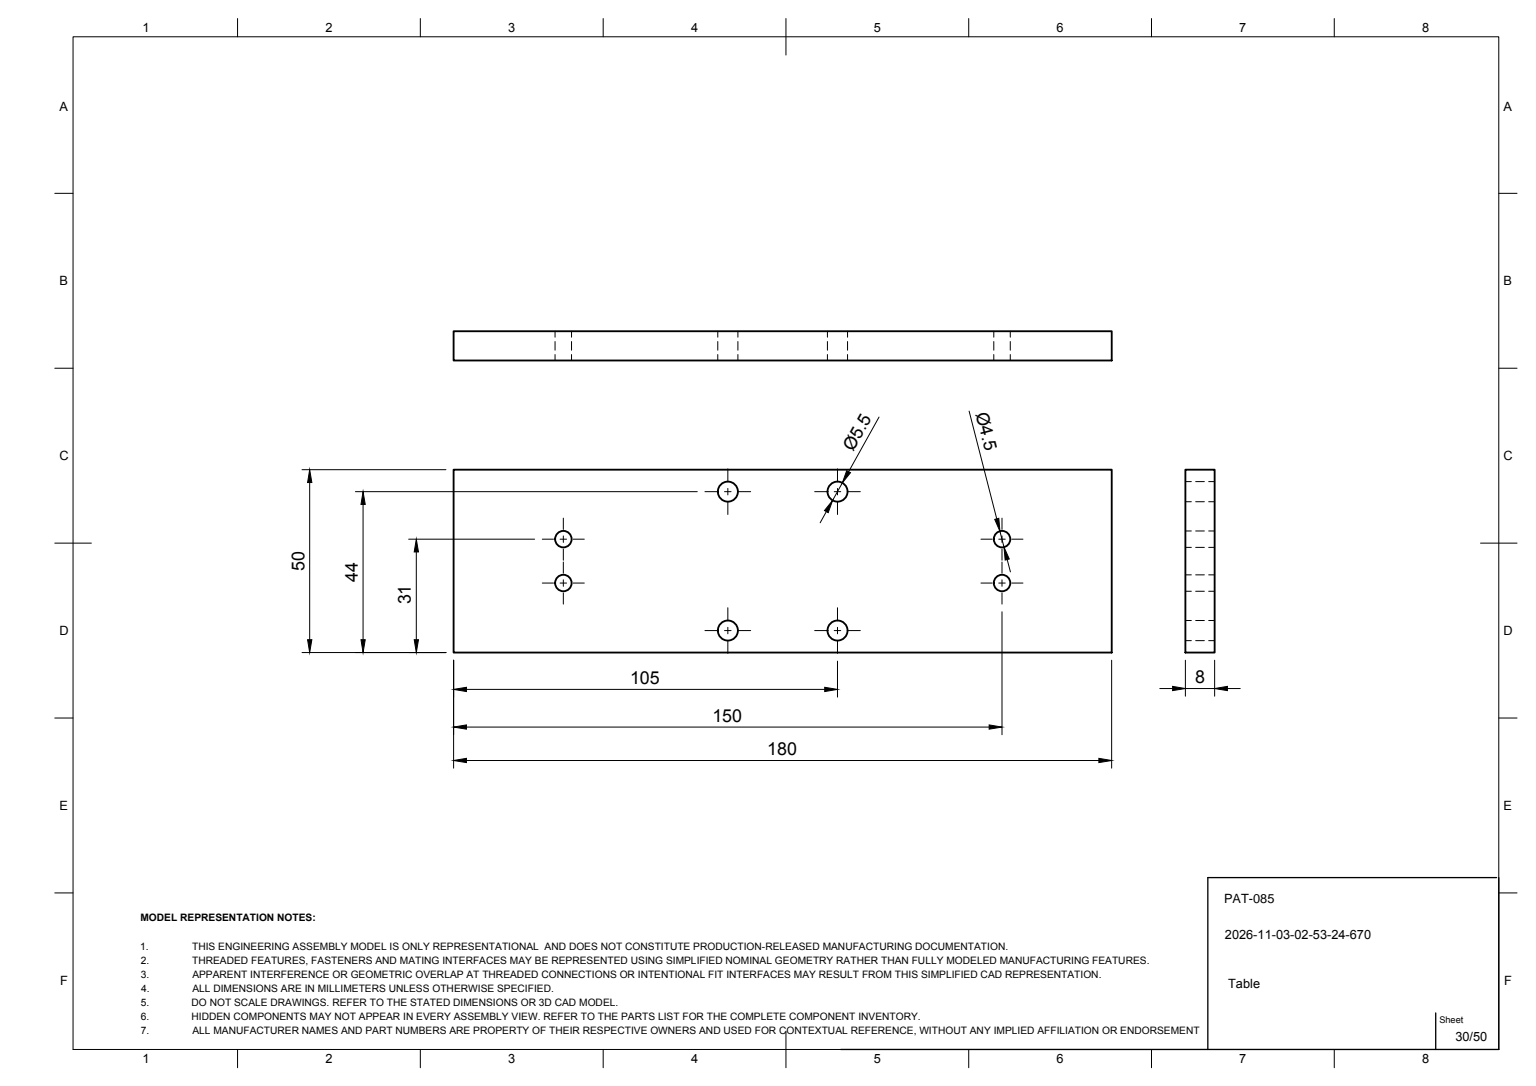
ISO-10303-21;
HEADER;
/* Generated by software containing ST-Developer
 * from STEP Tools, Inc. (www.steptools.com) 
 */

FILE_DESCRIPTION(
/* description */ ('Rack and pinion manual slide'),
/* implementation_level */ '2;1');

FILE_NAME(
/* name */ 'Table.step',
/* time_stamp */ '2026-10-28T03:22:49-07:00',
/* author */ (''),
/* organization */ (''),
/* preprocessor_version */ 'ST-DEVELOPER v20.2',
/* originating_system */ 'Autodesk Translation Framework v15.17.0.0',
/* authorisation */ '');

FILE_SCHEMA (('AUTOMOTIVE_DESIGN { 1 0 10303 214 3 1 1 }'));
ENDSEC;

DATA;
#10=MECHANICAL_DESIGN_GEOMETRIC_PRESENTATION_REPRESENTATION('',(#764),#34851);
#665=SHAPE_REPRESENTATION_RELATIONSHIP('SRR','None',#35102,#711);
#711=ADVANCED_BREP_SHAPE_REPRESENTATION('',(#815),#34827);
#764=STYLED_ITEM('',(#35425),#815);
#815=MANIFOLD_SOLID_BREP('Body1',#13786);
#985=FACE_BOUND('',#2766,.T.);
#986=FACE_BOUND('',#2767,.T.);
#987=FACE_BOUND('',#2768,.T.);
#988=FACE_BOUND('',#2769,.T.);
#989=FACE_BOUND('',#2770,.T.);
#990=FACE_BOUND('',#2771,.T.);
#991=FACE_BOUND('',#2772,.T.);
#992=FACE_BOUND('',#2773,.T.);
#993=FACE_BOUND('',#2775,.T.);
#994=FACE_BOUND('',#2776,.T.);
#995=FACE_BOUND('',#2777,.T.);
#996=FACE_BOUND('',#2778,.T.);
#997=FACE_BOUND('',#2779,.T.);
#998=FACE_BOUND('',#2780,.T.);
#999=FACE_BOUND('',#2781,.T.);
#1000=FACE_BOUND('',#2782,.T.);
#1245=PLANE('',#14956);
#1246=PLANE('',#14957);
#1247=PLANE('',#14958);
#1248=PLANE('',#14959);
#1249=PLANE('',#14960);
#1250=PLANE('',#14961);
#1862=FACE_OUTER_BOUND('',#2753,.T.);
#1863=FACE_OUTER_BOUND('',#2754,.T.);
#1864=FACE_OUTER_BOUND('',#2755,.T.);
#1865=FACE_OUTER_BOUND('',#2756,.T.);
#1866=FACE_OUTER_BOUND('',#2757,.T.);
#1867=FACE_OUTER_BOUND('',#2758,.T.);
#1868=FACE_OUTER_BOUND('',#2759,.T.);
#1869=FACE_OUTER_BOUND('',#2760,.T.);
#1870=FACE_OUTER_BOUND('',#2761,.T.);
#1871=FACE_OUTER_BOUND('',#2762,.T.);
#1872=FACE_OUTER_BOUND('',#2763,.T.);
#1873=FACE_OUTER_BOUND('',#2764,.T.);
#1874=FACE_OUTER_BOUND('',#2765,.T.);
#1875=FACE_OUTER_BOUND('',#2774,.T.);
#2753=EDGE_LOOP('',(#10748,#10749,#10750,#10751));
#2754=EDGE_LOOP('',(#10752,#10753,#10754,#10755));
#2755=EDGE_LOOP('',(#10756,#10757,#10758,#10759));
#2756=EDGE_LOOP('',(#10760,#10761,#10762,#10763));
#2757=EDGE_LOOP('',(#10764,#10765,#10766,#10767));
#2758=EDGE_LOOP('',(#10768,#10769,#10770,#10771));
#2759=EDGE_LOOP('',(#10772,#10773,#10774,#10775));
#2760=EDGE_LOOP('',(#10776,#10777,#10778,#10779));
#2761=EDGE_LOOP('',(#10780,#10781,#10782,#10783));
#2762=EDGE_LOOP('',(#10784,#10785,#10786,#10787));
#2763=EDGE_LOOP('',(#10788,#10789,#10790,#10791));
#2764=EDGE_LOOP('',(#10792,#10793,#10794,#10795));
#2765=EDGE_LOOP('',(#10796,#10797,#10798,#10799));
#2766=EDGE_LOOP('',(#10800));
#2767=EDGE_LOOP('',(#10801));
#2768=EDGE_LOOP('',(#10802));
#2769=EDGE_LOOP('',(#10803));
#2770=EDGE_LOOP('',(#10804));
#2771=EDGE_LOOP('',(#10805));
#2772=EDGE_LOOP('',(#10806));
#2773=EDGE_LOOP('',(#10807));
#2774=EDGE_LOOP('',(#10808,#10809,#10810,#10811));
#2775=EDGE_LOOP('',(#10812));
#2776=EDGE_LOOP('',(#10813));
#2777=EDGE_LOOP('',(#10814));
#2778=EDGE_LOOP('',(#10815));
#2779=EDGE_LOOP('',(#10816));
#2780=EDGE_LOOP('',(#10817));
#2781=EDGE_LOOP('',(#10818));
#2782=EDGE_LOOP('',(#10819));
#3714=LINE('',#21384,#5005);
#3715=LINE('',#21390,#5006);
#3716=LINE('',#21396,#5007);
#3717=LINE('',#21402,#5008);
#3718=LINE('',#21408,#5009);
#3719=LINE('',#21414,#5010);
#3720=LINE('',#21420,#5011);
#3721=LINE('',#21426,#5012);
#3722=LINE('',#21431,#5013);
#3723=LINE('',#21433,#5014);
#3724=LINE('',#21435,#5015);
#3725=LINE('',#21436,#5016);
#3726=LINE('',#21439,#5017);
#3727=LINE('',#21441,#5018);
#3728=LINE('',#21442,#5019);
#3729=LINE('',#21445,#5020);
#3730=LINE('',#21447,#5021);
#3731=LINE('',#21448,#5022);
#3732=LINE('',#21450,#5023);
#3733=LINE('',#21451,#5024);
#5005=VECTOR('',#17324,0.225000000000001);
#5006=VECTOR('',#17331,0.225);
#5007=VECTOR('',#17338,0.225);
#5008=VECTOR('',#17345,0.225000000000001);
#5009=VECTOR('',#17352,0.275);
#5010=VECTOR('',#17359,0.275);
#5011=VECTOR('',#17366,0.275);
#5012=VECTOR('',#17373,0.275);
#5013=VECTOR('',#17378,1.);
#5014=VECTOR('',#17379,1.);
#5015=VECTOR('',#17380,1.);
#5016=VECTOR('',#17381,1.);
#5017=VECTOR('',#17384,1.);
#5018=VECTOR('',#17385,1.);
#5019=VECTOR('',#17386,1.);
#5020=VECTOR('',#17389,1.);
#5021=VECTOR('',#17390,1.);
#5022=VECTOR('',#17391,1.);
#5023=VECTOR('',#17394,1.);
#5024=VECTOR('',#17395,1.);
#6057=CIRCLE('',#14933,0.225000000000001);
#6058=CIRCLE('',#14934,0.225000000000001);
#6059=CIRCLE('',#14936,0.225);
#6060=CIRCLE('',#14937,0.225);
#6061=CIRCLE('',#14939,0.225);
#6062=CIRCLE('',#14940,0.225);
#6063=CIRCLE('',#14942,0.225000000000001);
#6064=CIRCLE('',#14943,0.225000000000001);
#6065=CIRCLE('',#14945,0.275);
#6066=CIRCLE('',#14946,0.275);
#6067=CIRCLE('',#14948,0.275);
#6068=CIRCLE('',#14949,0.275);
#6069=CIRCLE('',#14951,0.275);
#6070=CIRCLE('',#14952,0.275);
#6071=CIRCLE('',#14954,0.275);
#6072=CIRCLE('',#14955,0.275);
#6734=VERTEX_POINT('',#21381);
#6735=VERTEX_POINT('',#21383);
#6736=VERTEX_POINT('',#21387);
#6737=VERTEX_POINT('',#21389);
#6738=VERTEX_POINT('',#21393);
#6739=VERTEX_POINT('',#21395);
#6740=VERTEX_POINT('',#21399);
#6741=VERTEX_POINT('',#21401);
#6742=VERTEX_POINT('',#21405);
#6743=VERTEX_POINT('',#21407);
#6744=VERTEX_POINT('',#21411);
#6745=VERTEX_POINT('',#21413);
#6746=VERTEX_POINT('',#21417);
#6747=VERTEX_POINT('',#21419);
#6748=VERTEX_POINT('',#21423);
#6749=VERTEX_POINT('',#21425);
#6750=VERTEX_POINT('',#21429);
#6751=VERTEX_POINT('',#21430);
#6752=VERTEX_POINT('',#21432);
#6753=VERTEX_POINT('',#21434);
#6754=VERTEX_POINT('',#21438);
#6755=VERTEX_POINT('',#21440);
#6756=VERTEX_POINT('',#21444);
#6757=VERTEX_POINT('',#21446);
#8186=EDGE_CURVE('',#6734,#6734,#6057,.T.);
#8187=EDGE_CURVE('',#6734,#6735,#3714,.T.);
#8188=EDGE_CURVE('',#6735,#6735,#6058,.T.);
#8189=EDGE_CURVE('',#6736,#6736,#6059,.T.);
#8190=EDGE_CURVE('',#6736,#6737,#3715,.T.);
#8191=EDGE_CURVE('',#6737,#6737,#6060,.T.);
#8192=EDGE_CURVE('',#6738,#6738,#6061,.T.);
#8193=EDGE_CURVE('',#6738,#6739,#3716,.T.);
#8194=EDGE_CURVE('',#6739,#6739,#6062,.T.);
#8195=EDGE_CURVE('',#6740,#6740,#6063,.T.);
#8196=EDGE_CURVE('',#6740,#6741,#3717,.T.);
#8197=EDGE_CURVE('',#6741,#6741,#6064,.T.);
#8198=EDGE_CURVE('',#6742,#6742,#6065,.T.);
#8199=EDGE_CURVE('',#6742,#6743,#3718,.T.);
#8200=EDGE_CURVE('',#6743,#6743,#6066,.T.);
#8201=EDGE_CURVE('',#6744,#6744,#6067,.T.);
#8202=EDGE_CURVE('',#6744,#6745,#3719,.T.);
#8203=EDGE_CURVE('',#6745,#6745,#6068,.T.);
#8204=EDGE_CURVE('',#6746,#6746,#6069,.T.);
#8205=EDGE_CURVE('',#6746,#6747,#3720,.T.);
#8206=EDGE_CURVE('',#6747,#6747,#6070,.T.);
#8207=EDGE_CURVE('',#6748,#6748,#6071,.T.);
#8208=EDGE_CURVE('',#6748,#6749,#3721,.T.);
#8209=EDGE_CURVE('',#6749,#6749,#6072,.T.);
#8210=EDGE_CURVE('',#6750,#6751,#3722,.T.);
#8211=EDGE_CURVE('',#6751,#6752,#3723,.T.);
#8212=EDGE_CURVE('',#6753,#6752,#3724,.T.);
#8213=EDGE_CURVE('',#6750,#6753,#3725,.T.);
#8214=EDGE_CURVE('',#6754,#6750,#3726,.T.);
#8215=EDGE_CURVE('',#6755,#6753,#3727,.T.);
#8216=EDGE_CURVE('',#6754,#6755,#3728,.T.);
#8217=EDGE_CURVE('',#6756,#6754,#3729,.T.);
#8218=EDGE_CURVE('',#6757,#6755,#3730,.T.);
#8219=EDGE_CURVE('',#6756,#6757,#3731,.T.);
#8220=EDGE_CURVE('',#6751,#6756,#3732,.T.);
#8221=EDGE_CURVE('',#6752,#6757,#3733,.T.);
#10748=ORIENTED_EDGE('',*,*,#8186,.F.);
#10749=ORIENTED_EDGE('',*,*,#8187,.T.);
#10750=ORIENTED_EDGE('',*,*,#8188,.F.);
#10751=ORIENTED_EDGE('',*,*,#8187,.F.);
#10752=ORIENTED_EDGE('',*,*,#8189,.F.);
#10753=ORIENTED_EDGE('',*,*,#8190,.T.);
#10754=ORIENTED_EDGE('',*,*,#8191,.F.);
#10755=ORIENTED_EDGE('',*,*,#8190,.F.);
#10756=ORIENTED_EDGE('',*,*,#8192,.F.);
#10757=ORIENTED_EDGE('',*,*,#8193,.T.);
#10758=ORIENTED_EDGE('',*,*,#8194,.F.);
#10759=ORIENTED_EDGE('',*,*,#8193,.F.);
#10760=ORIENTED_EDGE('',*,*,#8195,.F.);
#10761=ORIENTED_EDGE('',*,*,#8196,.T.);
#10762=ORIENTED_EDGE('',*,*,#8197,.F.);
#10763=ORIENTED_EDGE('',*,*,#8196,.F.);
#10764=ORIENTED_EDGE('',*,*,#8198,.F.);
#10765=ORIENTED_EDGE('',*,*,#8199,.T.);
#10766=ORIENTED_EDGE('',*,*,#8200,.F.);
#10767=ORIENTED_EDGE('',*,*,#8199,.F.);
#10768=ORIENTED_EDGE('',*,*,#8201,.F.);
#10769=ORIENTED_EDGE('',*,*,#8202,.T.);
#10770=ORIENTED_EDGE('',*,*,#8203,.F.);
#10771=ORIENTED_EDGE('',*,*,#8202,.F.);
#10772=ORIENTED_EDGE('',*,*,#8204,.F.);
#10773=ORIENTED_EDGE('',*,*,#8205,.T.);
#10774=ORIENTED_EDGE('',*,*,#8206,.F.);
#10775=ORIENTED_EDGE('',*,*,#8205,.F.);
#10776=ORIENTED_EDGE('',*,*,#8207,.F.);
#10777=ORIENTED_EDGE('',*,*,#8208,.T.);
#10778=ORIENTED_EDGE('',*,*,#8209,.F.);
#10779=ORIENTED_EDGE('',*,*,#8208,.F.);
#10780=ORIENTED_EDGE('',*,*,#8210,.T.);
#10781=ORIENTED_EDGE('',*,*,#8211,.T.);
#10782=ORIENTED_EDGE('',*,*,#8212,.F.);
#10783=ORIENTED_EDGE('',*,*,#8213,.F.);
#10784=ORIENTED_EDGE('',*,*,#8214,.T.);
#10785=ORIENTED_EDGE('',*,*,#8213,.T.);
#10786=ORIENTED_EDGE('',*,*,#8215,.F.);
#10787=ORIENTED_EDGE('',*,*,#8216,.F.);
#10788=ORIENTED_EDGE('',*,*,#8217,.T.);
#10789=ORIENTED_EDGE('',*,*,#8216,.T.);
#10790=ORIENTED_EDGE('',*,*,#8218,.F.);
#10791=ORIENTED_EDGE('',*,*,#8219,.F.);
#10792=ORIENTED_EDGE('',*,*,#8220,.T.);
#10793=ORIENTED_EDGE('',*,*,#8219,.T.);
#10794=ORIENTED_EDGE('',*,*,#8221,.F.);
#10795=ORIENTED_EDGE('',*,*,#8211,.F.);
#10796=ORIENTED_EDGE('',*,*,#8221,.T.);
#10797=ORIENTED_EDGE('',*,*,#8218,.T.);
#10798=ORIENTED_EDGE('',*,*,#8215,.T.);
#10799=ORIENTED_EDGE('',*,*,#8212,.T.);
#10800=ORIENTED_EDGE('',*,*,#8209,.T.);
#10801=ORIENTED_EDGE('',*,*,#8206,.T.);
#10802=ORIENTED_EDGE('',*,*,#8203,.T.);
#10803=ORIENTED_EDGE('',*,*,#8200,.T.);
#10804=ORIENTED_EDGE('',*,*,#8197,.T.);
#10805=ORIENTED_EDGE('',*,*,#8194,.T.);
#10806=ORIENTED_EDGE('',*,*,#8191,.T.);
#10807=ORIENTED_EDGE('',*,*,#8188,.T.);
#10808=ORIENTED_EDGE('',*,*,#8220,.F.);
#10809=ORIENTED_EDGE('',*,*,#8210,.F.);
#10810=ORIENTED_EDGE('',*,*,#8214,.F.);
#10811=ORIENTED_EDGE('',*,*,#8217,.F.);
#10812=ORIENTED_EDGE('',*,*,#8207,.T.);
#10813=ORIENTED_EDGE('',*,*,#8204,.T.);
#10814=ORIENTED_EDGE('',*,*,#8201,.T.);
#10815=ORIENTED_EDGE('',*,*,#8198,.T.);
#10816=ORIENTED_EDGE('',*,*,#8195,.T.);
#10817=ORIENTED_EDGE('',*,*,#8192,.T.);
#10818=ORIENTED_EDGE('',*,*,#8189,.T.);
#10819=ORIENTED_EDGE('',*,*,#8186,.T.);
#12942=CYLINDRICAL_SURFACE('',#14932,0.225000000000001);
#12943=CYLINDRICAL_SURFACE('',#14935,0.225);
#12944=CYLINDRICAL_SURFACE('',#14938,0.225);
#12945=CYLINDRICAL_SURFACE('',#14941,0.225000000000001);
#12946=CYLINDRICAL_SURFACE('',#14944,0.275);
#12947=CYLINDRICAL_SURFACE('',#14947,0.275);
#12948=CYLINDRICAL_SURFACE('',#14950,0.275);
#12949=CYLINDRICAL_SURFACE('',#14953,0.275);
#13340=ADVANCED_FACE('',(#1862),#12942,.F.);
#13341=ADVANCED_FACE('',(#1863),#12943,.F.);
#13342=ADVANCED_FACE('',(#1864),#12944,.F.);
#13343=ADVANCED_FACE('',(#1865),#12945,.F.);
#13344=ADVANCED_FACE('',(#1866),#12946,.F.);
#13345=ADVANCED_FACE('',(#1867),#12947,.F.);
#13346=ADVANCED_FACE('',(#1868),#12948,.F.);
#13347=ADVANCED_FACE('',(#1869),#12949,.F.);
#13348=ADVANCED_FACE('',(#1870),#1245,.T.);
#13349=ADVANCED_FACE('',(#1871),#1246,.T.);
#13350=ADVANCED_FACE('',(#1872),#1247,.T.);
#13351=ADVANCED_FACE('',(#1873),#1248,.T.);
#13352=ADVANCED_FACE('',(#1874,#985,#986,#987,#988,#989,#990,#991,#992),
#1249,.T.);
#13353=ADVANCED_FACE('',(#1875,#993,#994,#995,#996,#997,#998,#999,#1000),
#1250,.F.);
#13786=CLOSED_SHELL('',(#13340,#13341,#13342,#13343,#13344,#13345,#13346,
#13347,#13348,#13349,#13350,#13351,#13352,#13353));
#14931=AXIS2_PLACEMENT_3D('',#21379,#17318,#17319);
#14932=AXIS2_PLACEMENT_3D('',#21380,#17320,#17321);
#14933=AXIS2_PLACEMENT_3D('',#21382,#17322,#17323);
#14934=AXIS2_PLACEMENT_3D('',#21385,#17325,#17326);
#14935=AXIS2_PLACEMENT_3D('',#21386,#17327,#17328);
#14936=AXIS2_PLACEMENT_3D('',#21388,#17329,#17330);
#14937=AXIS2_PLACEMENT_3D('',#21391,#17332,#17333);
#14938=AXIS2_PLACEMENT_3D('',#21392,#17334,#17335);
#14939=AXIS2_PLACEMENT_3D('',#21394,#17336,#17337);
#14940=AXIS2_PLACEMENT_3D('',#21397,#17339,#17340);
#14941=AXIS2_PLACEMENT_3D('',#21398,#17341,#17342);
#14942=AXIS2_PLACEMENT_3D('',#21400,#17343,#17344);
#14943=AXIS2_PLACEMENT_3D('',#21403,#17346,#17347);
#14944=AXIS2_PLACEMENT_3D('',#21404,#17348,#17349);
#14945=AXIS2_PLACEMENT_3D('',#21406,#17350,#17351);
#14946=AXIS2_PLACEMENT_3D('',#21409,#17353,#17354);
#14947=AXIS2_PLACEMENT_3D('',#21410,#17355,#17356);
#14948=AXIS2_PLACEMENT_3D('',#21412,#17357,#17358);
#14949=AXIS2_PLACEMENT_3D('',#21415,#17360,#17361);
#14950=AXIS2_PLACEMENT_3D('',#21416,#17362,#17363);
#14951=AXIS2_PLACEMENT_3D('',#21418,#17364,#17365);
#14952=AXIS2_PLACEMENT_3D('',#21421,#17367,#17368);
#14953=AXIS2_PLACEMENT_3D('',#21422,#17369,#17370);
#14954=AXIS2_PLACEMENT_3D('',#21424,#17371,#17372);
#14955=AXIS2_PLACEMENT_3D('',#21427,#17374,#17375);
#14956=AXIS2_PLACEMENT_3D('',#21428,#17376,#17377);
#14957=AXIS2_PLACEMENT_3D('',#21437,#17382,#17383);
#14958=AXIS2_PLACEMENT_3D('',#21443,#17387,#17388);
#14959=AXIS2_PLACEMENT_3D('',#21449,#17392,#17393);
#14960=AXIS2_PLACEMENT_3D('',#21452,#17396,#17397);
#14961=AXIS2_PLACEMENT_3D('',#21453,#17398,#17399);
#17318=DIRECTION('axis',(0.,0.,1.));
#17319=DIRECTION('refdir',(1.,0.,0.));
#17320=DIRECTION('center_axis',(0.,0.,1.));
#17321=DIRECTION('ref_axis',(1.,0.,0.));
#17322=DIRECTION('center_axis',(0.,0.,1.));
#17323=DIRECTION('ref_axis',(1.,0.,0.));
#17324=DIRECTION('',(0.,0.,1.));
#17325=DIRECTION('center_axis',(0.,0.,-1.));
#17326=DIRECTION('ref_axis',(1.,0.,0.));
#17327=DIRECTION('center_axis',(0.,0.,1.));
#17328=DIRECTION('ref_axis',(1.,0.,0.));
#17329=DIRECTION('center_axis',(0.,0.,1.));
#17330=DIRECTION('ref_axis',(1.,0.,0.));
#17331=DIRECTION('',(0.,0.,1.));
#17332=DIRECTION('center_axis',(0.,0.,-1.));
#17333=DIRECTION('ref_axis',(1.,0.,0.));
#17334=DIRECTION('center_axis',(0.,0.,1.));
#17335=DIRECTION('ref_axis',(1.,0.,0.));
#17336=DIRECTION('center_axis',(0.,0.,1.));
#17337=DIRECTION('ref_axis',(1.,0.,0.));
#17338=DIRECTION('',(0.,0.,1.));
#17339=DIRECTION('center_axis',(0.,0.,-1.));
#17340=DIRECTION('ref_axis',(1.,0.,0.));
#17341=DIRECTION('center_axis',(0.,0.,1.));
#17342=DIRECTION('ref_axis',(1.,0.,0.));
#17343=DIRECTION('center_axis',(0.,0.,1.));
#17344=DIRECTION('ref_axis',(1.,0.,0.));
#17345=DIRECTION('',(0.,0.,1.));
#17346=DIRECTION('center_axis',(0.,0.,-1.));
#17347=DIRECTION('ref_axis',(1.,0.,0.));
#17348=DIRECTION('center_axis',(0.,0.,1.));
#17349=DIRECTION('ref_axis',(1.,0.,0.));
#17350=DIRECTION('center_axis',(0.,0.,1.));
#17351=DIRECTION('ref_axis',(1.,0.,0.));
#17352=DIRECTION('',(0.,0.,1.));
#17353=DIRECTION('center_axis',(0.,0.,-1.));
#17354=DIRECTION('ref_axis',(1.,0.,0.));
#17355=DIRECTION('center_axis',(0.,0.,1.));
#17356=DIRECTION('ref_axis',(1.,0.,0.));
#17357=DIRECTION('center_axis',(0.,0.,1.));
#17358=DIRECTION('ref_axis',(1.,0.,0.));
#17359=DIRECTION('',(0.,0.,1.));
#17360=DIRECTION('center_axis',(0.,0.,-1.));
#17361=DIRECTION('ref_axis',(1.,0.,0.));
#17362=DIRECTION('center_axis',(0.,0.,1.));
#17363=DIRECTION('ref_axis',(1.,0.,0.));
#17364=DIRECTION('center_axis',(0.,0.,1.));
#17365=DIRECTION('ref_axis',(1.,0.,0.));
#17366=DIRECTION('',(0.,0.,1.));
#17367=DIRECTION('center_axis',(0.,0.,-1.));
#17368=DIRECTION('ref_axis',(1.,0.,0.));
#17369=DIRECTION('center_axis',(0.,0.,1.));
#17370=DIRECTION('ref_axis',(1.,0.,0.));
#17371=DIRECTION('center_axis',(0.,0.,1.));
#17372=DIRECTION('ref_axis',(1.,0.,0.));
#17373=DIRECTION('',(0.,0.,1.));
#17374=DIRECTION('center_axis',(0.,0.,-1.));
#17375=DIRECTION('ref_axis',(1.,0.,0.));
#17376=DIRECTION('center_axis',(0.,1.,0.));
#17377=DIRECTION('ref_axis',(-1.,0.,0.));
#17378=DIRECTION('',(-1.,0.,0.));
#17379=DIRECTION('',(0.,0.,1.));
#17380=DIRECTION('',(-1.,0.,0.));
#17381=DIRECTION('',(0.,0.,1.));
#17382=DIRECTION('center_axis',(1.,0.,0.));
#17383=DIRECTION('ref_axis',(0.,1.,0.));
#17384=DIRECTION('',(0.,1.,0.));
#17385=DIRECTION('',(0.,1.,0.));
#17386=DIRECTION('',(0.,0.,1.));
#17387=DIRECTION('center_axis',(0.,-1.,0.));
#17388=DIRECTION('ref_axis',(1.,0.,0.));
#17389=DIRECTION('',(1.,0.,0.));
#17390=DIRECTION('',(1.,0.,0.));
#17391=DIRECTION('',(0.,0.,1.));
#17392=DIRECTION('center_axis',(-1.,0.,0.));
#17393=DIRECTION('ref_axis',(0.,-1.,0.));
#17394=DIRECTION('',(0.,-1.,0.));
#17395=DIRECTION('',(0.,-1.,0.));
#17396=DIRECTION('center_axis',(0.,0.,1.));
#17397=DIRECTION('ref_axis',(1.,0.,0.));
#17398=DIRECTION('center_axis',(0.,0.,1.));
#17399=DIRECTION('ref_axis',(1.,0.,0.));
#21379=CARTESIAN_POINT('',(0.,0.,0.));
#21380=CARTESIAN_POINT('Origin',(17.,-0.6,6.1));
#21381=CARTESIAN_POINT('',(16.775,-0.6,6.2));
#21382=CARTESIAN_POINT('Origin',(17.,-0.6,6.2));
#21383=CARTESIAN_POINT('',(16.775,-0.6,7.));
#21384=CARTESIAN_POINT('',(16.775,-0.6,6.1));
#21385=CARTESIAN_POINT('Origin',(17.,-0.6,7.));
#21386=CARTESIAN_POINT('Origin',(5.,0.6,6.1));
#21387=CARTESIAN_POINT('',(4.775,0.6,6.2));
#21388=CARTESIAN_POINT('Origin',(5.,0.6,6.2));
#21389=CARTESIAN_POINT('',(4.775,0.6,7.));
#21390=CARTESIAN_POINT('',(4.775,0.6,6.1));
#21391=CARTESIAN_POINT('Origin',(5.,0.6,7.));
#21392=CARTESIAN_POINT('Origin',(5.,-0.6,6.1));
#21393=CARTESIAN_POINT('',(4.775,-0.6,6.2));
#21394=CARTESIAN_POINT('Origin',(5.,-0.6,6.2));
#21395=CARTESIAN_POINT('',(4.775,-0.6,7.));
#21396=CARTESIAN_POINT('',(4.775,-0.6,6.1));
#21397=CARTESIAN_POINT('Origin',(5.,-0.6,7.));
#21398=CARTESIAN_POINT('Origin',(17.,0.6,6.1));
#21399=CARTESIAN_POINT('',(16.775,0.6,6.2));
#21400=CARTESIAN_POINT('Origin',(17.,0.6,6.2));
#21401=CARTESIAN_POINT('',(16.775,0.6,7.));
#21402=CARTESIAN_POINT('',(16.775,0.6,6.1));
#21403=CARTESIAN_POINT('Origin',(17.,0.6,7.));
#21404=CARTESIAN_POINT('Origin',(12.5,-1.9,6.1));
#21405=CARTESIAN_POINT('',(12.225,-1.9,6.2));
#21406=CARTESIAN_POINT('Origin',(12.5,-1.9,6.2));
#21407=CARTESIAN_POINT('',(12.225,-1.9,7.));
#21408=CARTESIAN_POINT('',(12.225,-1.9,6.1));
#21409=CARTESIAN_POINT('Origin',(12.5,-1.9,7.));
#21410=CARTESIAN_POINT('Origin',(9.5,1.9,6.1));
#21411=CARTESIAN_POINT('',(9.225,1.9,6.2));
#21412=CARTESIAN_POINT('Origin',(9.5,1.9,6.2));
#21413=CARTESIAN_POINT('',(9.225,1.9,7.));
#21414=CARTESIAN_POINT('',(9.225,1.9,6.1));
#21415=CARTESIAN_POINT('Origin',(9.5,1.9,7.));
#21416=CARTESIAN_POINT('Origin',(9.5,-1.9,6.1));
#21417=CARTESIAN_POINT('',(9.225,-1.9,6.2));
#21418=CARTESIAN_POINT('Origin',(9.5,-1.9,6.2));
#21419=CARTESIAN_POINT('',(9.225,-1.9,7.));
#21420=CARTESIAN_POINT('',(9.225,-1.9,6.1));
#21421=CARTESIAN_POINT('Origin',(9.5,-1.9,7.));
#21422=CARTESIAN_POINT('Origin',(12.5,1.9,6.1));
#21423=CARTESIAN_POINT('',(12.225,1.9,6.2));
#21424=CARTESIAN_POINT('Origin',(12.5,1.9,6.2));
#21425=CARTESIAN_POINT('',(12.225,1.9,7.));
#21426=CARTESIAN_POINT('',(12.225,1.9,6.1));
#21427=CARTESIAN_POINT('Origin',(12.5,1.9,7.));
#21428=CARTESIAN_POINT('Origin',(20.,2.5,6.2));
#21429=CARTESIAN_POINT('',(20.,2.5,6.2));
#21430=CARTESIAN_POINT('',(2.,2.5,6.2));
#21431=CARTESIAN_POINT('',(20.,2.5,6.2));
#21432=CARTESIAN_POINT('',(2.,2.5,7.));
#21433=CARTESIAN_POINT('',(2.,2.5,6.2));
#21434=CARTESIAN_POINT('',(20.,2.5,7.));
#21435=CARTESIAN_POINT('',(20.,2.5,7.));
#21436=CARTESIAN_POINT('',(20.,2.5,6.2));
#21437=CARTESIAN_POINT('Origin',(20.,-2.5,6.2));
#21438=CARTESIAN_POINT('',(20.,-2.5,6.2));
#21439=CARTESIAN_POINT('',(20.,-2.5,6.2));
#21440=CARTESIAN_POINT('',(20.,-2.5,7.));
#21441=CARTESIAN_POINT('',(20.,-2.5,7.));
#21442=CARTESIAN_POINT('',(20.,-2.5,6.2));
#21443=CARTESIAN_POINT('Origin',(2.,-2.5,6.2));
#21444=CARTESIAN_POINT('',(2.,-2.5,6.2));
#21445=CARTESIAN_POINT('',(2.,-2.5,6.2));
#21446=CARTESIAN_POINT('',(2.,-2.5,7.));
#21447=CARTESIAN_POINT('',(2.,-2.5,7.));
#21448=CARTESIAN_POINT('',(2.,-2.5,6.2));
#21449=CARTESIAN_POINT('Origin',(2.,2.5,6.2));
#21450=CARTESIAN_POINT('',(2.,2.5,6.2));
#21451=CARTESIAN_POINT('',(2.,2.5,7.));
#21452=CARTESIAN_POINT('Origin',(11.,0.,7.));
#21453=CARTESIAN_POINT('Origin',(11.,0.,6.2));
#34773=UNCERTAINTY_MEASURE_WITH_UNIT(LENGTH_MEASURE(0.001),#34852,
'DISTANCE_ACCURACY_VALUE',
'Maximum model space distance between geometric entities at asserted c
onnectivities');
#34797=UNCERTAINTY_MEASURE_WITH_UNIT(LENGTH_MEASURE(0.001),#34852,
'DISTANCE_ACCURACY_VALUE',
'Maximum model space distance between geometric entities at asserted c
onnectivities');
#34827=(
GEOMETRIC_REPRESENTATION_CONTEXT(3)
GLOBAL_UNCERTAINTY_ASSIGNED_CONTEXT((#34773))
GLOBAL_UNIT_ASSIGNED_CONTEXT((#34852,#34854,#34855))
REPRESENTATION_CONTEXT('','3D')
);
#34851=(
GEOMETRIC_REPRESENTATION_CONTEXT(3)
GLOBAL_UNCERTAINTY_ASSIGNED_CONTEXT((#34797))
GLOBAL_UNIT_ASSIGNED_CONTEXT((#34852,#34854,#34855))
REPRESENTATION_CONTEXT('','3D')
);
#34852=(
LENGTH_UNIT()
NAMED_UNIT(*)
SI_UNIT(.CENTI.,.METRE.)
);
#34854=(
NAMED_UNIT(*)
PLANE_ANGLE_UNIT()
SI_UNIT($,.RADIAN.)
);
#34855=(
NAMED_UNIT(*)
SI_UNIT($,.STERADIAN.)
SOLID_ANGLE_UNIT()
);
#34885=SHAPE_DEFINITION_REPRESENTATION(#34943,#35102);
#34943=PRODUCT_DEFINITION_SHAPE('',$,#35156);
#35102=SHAPE_REPRESENTATION('',(#14931),#34827);
#35126=PRODUCT_DEFINITION_CONTEXT('part definition',#35287,'design');
#35156=PRODUCT_DEFINITION('Table','Table',#35209,#35126);
#35209=PRODUCT_DEFINITION_FORMATION('',$,#35318);
#35287=APPLICATION_CONTEXT(
'Core Data for Automotive Mechanical Design Process');
#35288=PRODUCT_CONTEXT('part definition',#35287,'mechanical');
#35318=PRODUCT('Table','Table','Table',(#35288));
#35419=COLOUR_RGB('Off White',0.89,0.88,0.83);
#35420=FILL_AREA_STYLE_COLOUR('',#35419);
#35421=FILL_AREA_STYLE('',(#35420));
#35422=SURFACE_STYLE_FILL_AREA(#35421);
#35423=SURFACE_SIDE_STYLE('',(#35422));
#35424=SURFACE_STYLE_USAGE(.BOTH.,#35423);
#35425=PRESENTATION_STYLE_ASSIGNMENT((#35424));
ENDSEC;
END-ISO-10303-21;
